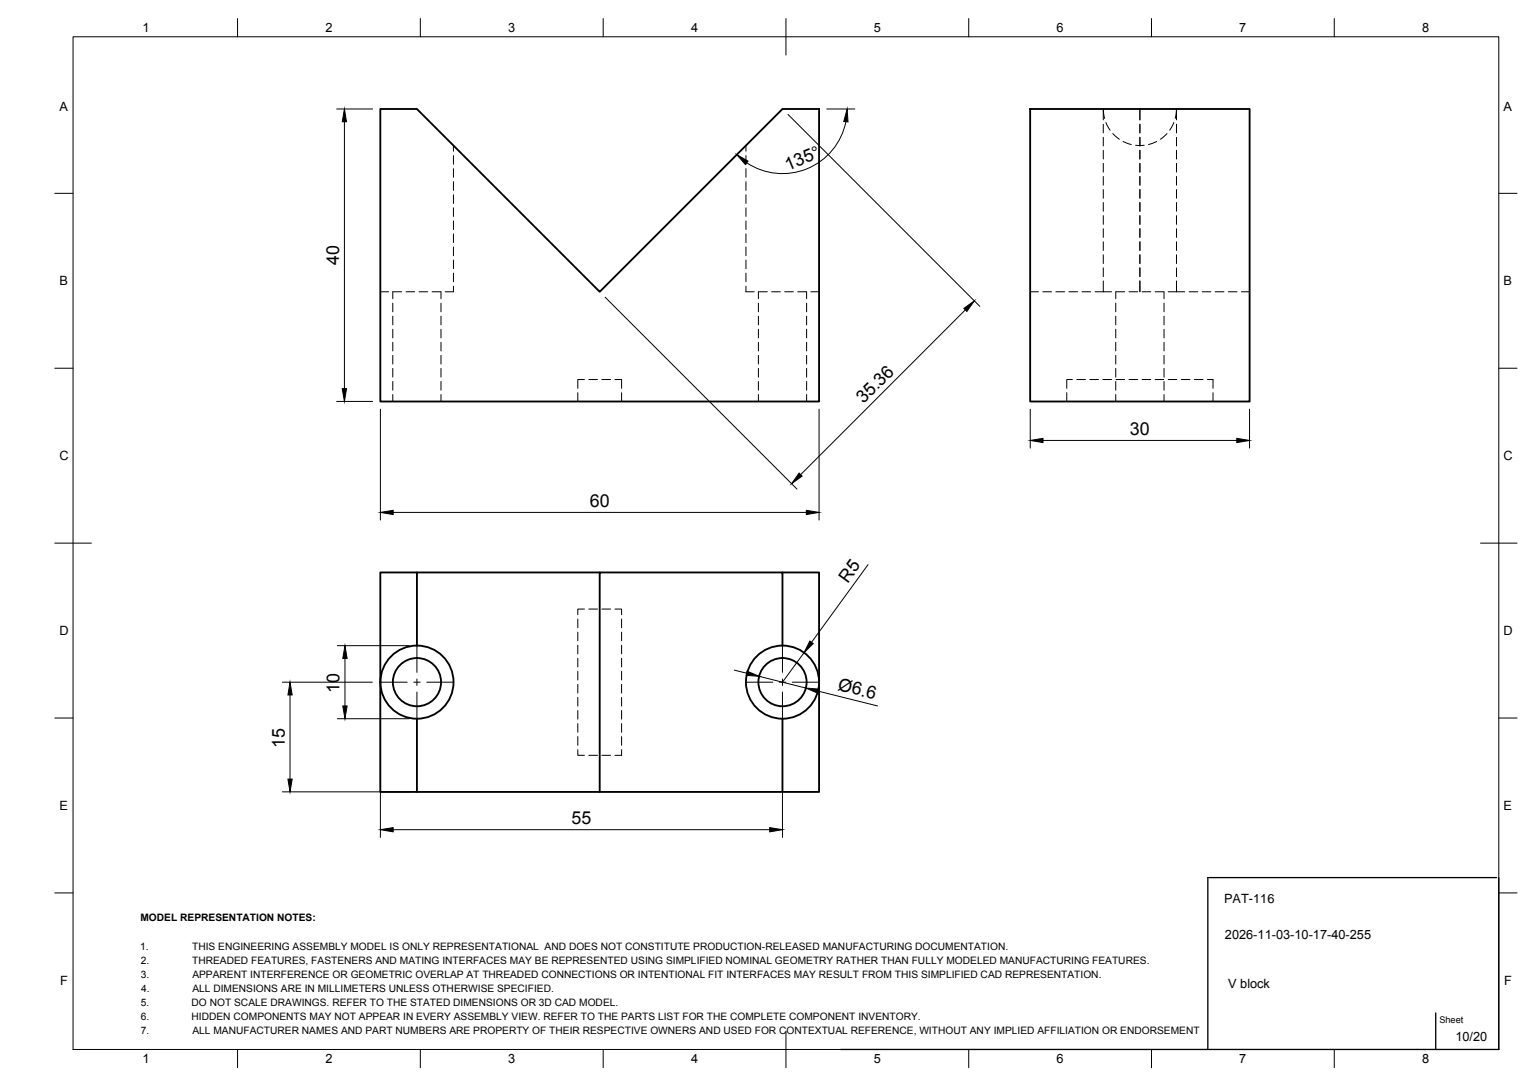
ISO-10303-21;
HEADER;
/* Generated by software containing ST-Developer
 * from STEP Tools, Inc. (www.steptools.com) 
 */

FILE_DESCRIPTION(
/* description */ ('V-block with clamp strap'),
/* implementation_level */ '2;1');

FILE_NAME(
/* name */ 'V block.step',
/* time_stamp */ '2026-10-27T10:50:53-07:00',
/* author */ (''),
/* organization */ (''),
/* preprocessor_version */ 'ST-DEVELOPER v20.2',
/* originating_system */ 'Autodesk Translation Framework v15.17.0.0',
/* authorisation */ '');

FILE_SCHEMA (('AUTOMOTIVE_DESIGN { 1 0 10303 214 3 1 1 }'));
ENDSEC;

DATA;
#10=MECHANICAL_DESIGN_GEOMETRIC_PRESENTATION_REPRESENTATION('',(#271),#7344);
#220=ELLIPSE('',#4506,0.707106781186547,0.5);
#221=ELLIPSE('',#4518,0.707106781186547,0.5);
#229=SHAPE_REPRESENTATION_RELATIONSHIP('SRR','None',#7447,#250);
#250=ADVANCED_BREP_SHAPE_REPRESENTATION('',(#292),#7326);
#271=STYLED_ITEM('',(#7610),#292);
#292=MANIFOLD_SOLID_BREP('Body1',#4153);
#339=FACE_BOUND('',#901,.T.);
#340=FACE_BOUND('',#904,.T.);
#341=FACE_BOUND('',#918,.T.);
#342=FACE_BOUND('',#919,.T.);
#343=FACE_BOUND('',#920,.T.);
#408=CIRCLE('',#4501,0.5);
#409=CIRCLE('',#4502,0.5);
#410=CIRCLE('',#4504,0.5);
#411=CIRCLE('',#4505,0.5);
#412=CIRCLE('',#4513,0.5);
#413=CIRCLE('',#4514,0.5);
#414=CIRCLE('',#4516,0.33);
#415=CIRCLE('',#4519,0.5);
#416=CIRCLE('',#4520,0.5);
#417=CIRCLE('',#4522,0.33);
#418=CIRCLE('',#4528,0.33);
#419=CIRCLE('',#4530,0.33);
#521=CYLINDRICAL_SURFACE('',#4500,0.5);
#522=CYLINDRICAL_SURFACE('',#4503,0.5);
#523=CYLINDRICAL_SURFACE('',#4512,0.5);
#524=CYLINDRICAL_SURFACE('',#4517,0.5);
#525=CYLINDRICAL_SURFACE('',#4527,0.33);
#526=CYLINDRICAL_SURFACE('',#4529,0.33);
#618=FACE_OUTER_BOUND('',#892,.T.);
#619=FACE_OUTER_BOUND('',#893,.T.);
#620=FACE_OUTER_BOUND('',#894,.T.);
#621=FACE_OUTER_BOUND('',#895,.T.);
#622=FACE_OUTER_BOUND('',#896,.T.);
#623=FACE_OUTER_BOUND('',#897,.T.);
#624=FACE_OUTER_BOUND('',#898,.T.);
#625=FACE_OUTER_BOUND('',#899,.T.);
#626=FACE_OUTER_BOUND('',#900,.T.);
#627=FACE_OUTER_BOUND('',#902,.T.);
#628=FACE_OUTER_BOUND('',#903,.T.);
#629=FACE_OUTER_BOUND('',#905,.T.);
#630=FACE_OUTER_BOUND('',#906,.T.);
#631=FACE_OUTER_BOUND('',#907,.T.);
#632=FACE_OUTER_BOUND('',#908,.T.);
#633=FACE_OUTER_BOUND('',#909,.T.);
#634=FACE_OUTER_BOUND('',#910,.T.);
#635=FACE_OUTER_BOUND('',#911,.T.);
#636=FACE_OUTER_BOUND('',#912,.T.);
#637=FACE_OUTER_BOUND('',#913,.T.);
#638=FACE_OUTER_BOUND('',#914,.T.);
#639=FACE_OUTER_BOUND('',#915,.T.);
#640=FACE_OUTER_BOUND('',#916,.T.);
#641=FACE_OUTER_BOUND('',#917,.T.);
#892=EDGE_LOOP('',(#2960,#2961,#2962,#2963));
#893=EDGE_LOOP('',(#2964,#2965,#2966,#2967,#2968));
#894=EDGE_LOOP('',(#2969,#2970,#2971,#2972));
#895=EDGE_LOOP('',(#2973,#2974,#2975,#2976));
#896=EDGE_LOOP('',(#2977,#2978,#2979,#2980));
#897=EDGE_LOOP('',(#2981,#2982,#2983,#2984));
#898=EDGE_LOOP('',(#2985,#2986,#2987,#2988));
#899=EDGE_LOOP('',(#2989,#2990,#2991,#2992));
#900=EDGE_LOOP('',(#2993,#2994));
#901=EDGE_LOOP('',(#2995));
#902=EDGE_LOOP('',(#2996,#2997,#2998,#2999,#3000));
#903=EDGE_LOOP('',(#3001,#3002));
#904=EDGE_LOOP('',(#3003));
#905=EDGE_LOOP('',(#3004,#3005,#3006,#3007,#3008,#3009));
#906=EDGE_LOOP('',(#3010,#3011,#3012,#3013));
#907=EDGE_LOOP('',(#3014,#3015,#3016,#3017,#3018,#3019));
#908=EDGE_LOOP('',(#3020,#3021,#3022,#3023));
#909=EDGE_LOOP('',(#3024,#3025,#3026,#3027));
#910=EDGE_LOOP('',(#3028,#3029,#3030,#3031));
#911=EDGE_LOOP('',(#3032,#3033,#3034,#3035));
#912=EDGE_LOOP('',(#3036,#3037,#3038,#3039));
#913=EDGE_LOOP('',(#3040,#3041,#3042,#3043,#3044,#3045,#3046));
#914=EDGE_LOOP('',(#3047,#3048,#3049,#3050,#3051,#3052,#3053));
#915=EDGE_LOOP('',(#3054,#3055,#3056,#3057,#3058,#3059,#3060));
#916=EDGE_LOOP('',(#3061,#3062,#3063,#3064,#3065,#3066,#3067));
#917=EDGE_LOOP('',(#3068,#3069,#3070,#3071));
#918=EDGE_LOOP('',(#3072,#3073,#3074,#3075));
#919=EDGE_LOOP('',(#3076));
#920=EDGE_LOOP('',(#3077));
#1213=LINE('',#6373,#1578);
#1214=LINE('',#6377,#1579);
#1215=LINE('',#6382,#1580);
#1216=LINE('',#6386,#1581);
#1217=LINE('',#6393,#1582);
#1218=LINE('',#6395,#1583);
#1219=LINE('',#6397,#1584);
#1220=LINE('',#6398,#1585);
#1221=LINE('',#6401,#1586);
#1222=LINE('',#6403,#1587);
#1223=LINE('',#6404,#1588);
#1224=LINE('',#6407,#1589);
#1225=LINE('',#6409,#1590);
#1226=LINE('',#6410,#1591);
#1227=LINE('',#6412,#1592);
#1228=LINE('',#6413,#1593);
#1229=LINE('',#6417,#1594);
#1230=LINE('',#6426,#1595);
#1231=LINE('',#6433,#1596);
#1232=LINE('',#6435,#1597);
#1233=LINE('',#6437,#1598);
#1234=LINE('',#6439,#1599);
#1235=LINE('',#6440,#1600);
#1236=LINE('',#6443,#1601);
#1237=LINE('',#6444,#1602);
#1238=LINE('',#6447,#1603);
#1239=LINE('',#6448,#1604);
#1240=LINE('',#6450,#1605);
#1241=LINE('',#6451,#1606);
#1242=LINE('',#6454,#1607);
#1243=LINE('',#6455,#1608);
#1244=LINE('',#6459,#1609);
#1245=LINE('',#6463,#1610);
#1246=LINE('',#6466,#1611);
#1247=LINE('',#6467,#1612);
#1248=LINE('',#6470,#1613);
#1249=LINE('',#6471,#1614);
#1250=LINE('',#6474,#1615);
#1251=LINE('',#6476,#1616);
#1252=LINE('',#6477,#1617);
#1253=LINE('',#6480,#1618);
#1254=LINE('',#6481,#1619);
#1255=LINE('',#6484,#1620);
#1256=LINE('',#6485,#1621);
#1257=LINE('',#6487,#1622);
#1578=VECTOR('',#5137,0.5);
#1579=VECTOR('',#5140,1.);
#1580=VECTOR('',#5145,0.5);
#1581=VECTOR('',#5148,1.);
#1582=VECTOR('',#5155,1.);
#1583=VECTOR('',#5156,1.);
#1584=VECTOR('',#5157,1.);
#1585=VECTOR('',#5158,1.);
#1586=VECTOR('',#5161,1.);
#1587=VECTOR('',#5162,1.);
#1588=VECTOR('',#5163,1.);
#1589=VECTOR('',#5166,1.);
#1590=VECTOR('',#5167,1.);
#1591=VECTOR('',#5168,1.);
#1592=VECTOR('',#5171,1.);
#1593=VECTOR('',#5172,1.);
#1594=VECTOR('',#5179,1.);
#1595=VECTOR('',#5192,1.);
#1596=VECTOR('',#5201,1.);
#1597=VECTOR('',#5202,1.);
#1598=VECTOR('',#5203,1.);
#1599=VECTOR('',#5204,1.);
#1600=VECTOR('',#5205,1.);
#1601=VECTOR('',#5208,1.);
#1602=VECTOR('',#5209,1.);
#1603=VECTOR('',#5212,1.);
#1604=VECTOR('',#5213,1.);
#1605=VECTOR('',#5214,1.);
#1606=VECTOR('',#5215,1.);
#1607=VECTOR('',#5218,1.);
#1608=VECTOR('',#5219,1.);
#1609=VECTOR('',#5224,0.33);
#1610=VECTOR('',#5229,0.33);
#1611=VECTOR('',#5232,1.);
#1612=VECTOR('',#5233,1.);
#1613=VECTOR('',#5236,1.);
#1614=VECTOR('',#5237,1.);
#1615=VECTOR('',#5240,1.);
#1616=VECTOR('',#5241,1.);
#1617=VECTOR('',#5242,1.);
#1618=VECTOR('',#5245,1.);
#1619=VECTOR('',#5246,1.);
#1620=VECTOR('',#5249,1.);
#1621=VECTOR('',#5250,1.);
#1622=VECTOR('',#5253,1.);
#1931=VERTEX_POINT('',#6371);
#1932=VERTEX_POINT('',#6372);
#1933=VERTEX_POINT('',#6374);
#1934=VERTEX_POINT('',#6376);
#1935=VERTEX_POINT('',#6380);
#1936=VERTEX_POINT('',#6381);
#1937=VERTEX_POINT('',#6383);
#1938=VERTEX_POINT('',#6385);
#1939=VERTEX_POINT('',#6387);
#1940=VERTEX_POINT('',#6391);
#1941=VERTEX_POINT('',#6392);
#1942=VERTEX_POINT('',#6394);
#1943=VERTEX_POINT('',#6396);
#1944=VERTEX_POINT('',#6400);
#1945=VERTEX_POINT('',#6402);
#1946=VERTEX_POINT('',#6406);
#1947=VERTEX_POINT('',#6408);
#1948=VERTEX_POINT('',#6420);
#1949=VERTEX_POINT('',#6423);
#1950=VERTEX_POINT('',#6429);
#1951=VERTEX_POINT('',#6432);
#1952=VERTEX_POINT('',#6434);
#1953=VERTEX_POINT('',#6436);
#1954=VERTEX_POINT('',#6438);
#1955=VERTEX_POINT('',#6442);
#1956=VERTEX_POINT('',#6446);
#1957=VERTEX_POINT('',#6449);
#1958=VERTEX_POINT('',#6453);
#1959=VERTEX_POINT('',#6457);
#1960=VERTEX_POINT('',#6461);
#1961=VERTEX_POINT('',#6465);
#1962=VERTEX_POINT('',#6469);
#1963=VERTEX_POINT('',#6473);
#1964=VERTEX_POINT('',#6475);
#1965=VERTEX_POINT('',#6479);
#1966=VERTEX_POINT('',#6483);
#2306=EDGE_CURVE('',#1931,#1932,#1213,.T.);
#2307=EDGE_CURVE('',#1933,#1931,#408,.T.);
#2308=EDGE_CURVE('',#1933,#1934,#1214,.T.);
#2309=EDGE_CURVE('',#1932,#1934,#409,.T.);
#2310=EDGE_CURVE('',#1935,#1936,#1215,.T.);
#2311=EDGE_CURVE('',#1937,#1935,#410,.T.);
#2312=EDGE_CURVE('',#1937,#1938,#1216,.T.);
#2313=EDGE_CURVE('',#1939,#1938,#411,.T.);
#2314=EDGE_CURVE('',#1936,#1939,#220,.T.);
#2315=EDGE_CURVE('',#1940,#1941,#1217,.T.);
#2316=EDGE_CURVE('',#1940,#1942,#1218,.T.);
#2317=EDGE_CURVE('',#1942,#1943,#1219,.T.);
#2318=EDGE_CURVE('',#1941,#1943,#1220,.T.);
#2319=EDGE_CURVE('',#1941,#1944,#1221,.T.);
#2320=EDGE_CURVE('',#1943,#1945,#1222,.T.);
#2321=EDGE_CURVE('',#1944,#1945,#1223,.T.);
#2322=EDGE_CURVE('',#1944,#1946,#1224,.T.);
#2323=EDGE_CURVE('',#1945,#1947,#1225,.T.);
#2324=EDGE_CURVE('',#1946,#1947,#1226,.T.);
#2325=EDGE_CURVE('',#1946,#1940,#1227,.T.);
#2326=EDGE_CURVE('',#1947,#1942,#1228,.T.);
#2327=EDGE_CURVE('',#1938,#1936,#412,.T.);
#2328=EDGE_CURVE('',#1937,#1938,#1229,.T.);
#2329=EDGE_CURVE('',#1935,#1937,#413,.T.);
#2330=EDGE_CURVE('',#1948,#1948,#414,.T.);
#2331=EDGE_CURVE('',#1949,#1932,#221,.T.);
#2332=EDGE_CURVE('',#1934,#1949,#415,.T.);
#2333=EDGE_CURVE('',#1933,#1934,#1230,.T.);
#2334=EDGE_CURVE('',#1931,#1933,#416,.T.);
#2335=EDGE_CURVE('',#1950,#1950,#417,.T.);
#2336=EDGE_CURVE('',#1951,#1939,#1231,.T.);
#2337=EDGE_CURVE('',#1952,#1951,#1232,.T.);
#2338=EDGE_CURVE('',#1953,#1952,#1233,.T.);
#2339=EDGE_CURVE('',#1954,#1953,#1234,.T.);
#2340=EDGE_CURVE('',#1936,#1954,#1235,.T.);
#2341=EDGE_CURVE('',#1938,#1955,#1236,.T.);
#2342=EDGE_CURVE('',#1955,#1951,#1237,.T.);
#2343=EDGE_CURVE('',#1956,#1932,#1238,.T.);
#2344=EDGE_CURVE('',#1953,#1956,#1239,.T.);
#2345=EDGE_CURVE('',#1957,#1952,#1240,.T.);
#2346=EDGE_CURVE('',#1949,#1957,#1241,.T.);
#2347=EDGE_CURVE('',#1934,#1958,#1242,.T.);
#2348=EDGE_CURVE('',#1958,#1956,#1243,.T.);
#2349=EDGE_CURVE('',#1959,#1959,#418,.T.);
#2350=EDGE_CURVE('',#1959,#1948,#1244,.T.);
#2351=EDGE_CURVE('',#1960,#1960,#419,.T.);
#2352=EDGE_CURVE('',#1960,#1950,#1245,.T.);
#2353=EDGE_CURVE('',#1954,#1961,#1246,.T.);
#2354=EDGE_CURVE('',#1961,#1938,#1247,.T.);
#2355=EDGE_CURVE('',#1957,#1962,#1248,.T.);
#2356=EDGE_CURVE('',#1962,#1934,#1249,.T.);
#2357=EDGE_CURVE('',#1963,#1958,#1250,.T.);
#2358=EDGE_CURVE('',#1963,#1964,#1251,.T.);
#2359=EDGE_CURVE('',#1964,#1961,#1252,.T.);
#2360=EDGE_CURVE('',#1965,#1963,#1253,.T.);
#2361=EDGE_CURVE('',#1965,#1962,#1254,.T.);
#2362=EDGE_CURVE('',#1966,#1955,#1255,.T.);
#2363=EDGE_CURVE('',#1966,#1965,#1256,.T.);
#2364=EDGE_CURVE('',#1964,#1966,#1257,.T.);
#2960=ORIENTED_EDGE('',*,*,#2306,.F.);
#2961=ORIENTED_EDGE('',*,*,#2307,.F.);
#2962=ORIENTED_EDGE('',*,*,#2308,.T.);
#2963=ORIENTED_EDGE('',*,*,#2309,.F.);
#2964=ORIENTED_EDGE('',*,*,#2310,.F.);
#2965=ORIENTED_EDGE('',*,*,#2311,.F.);
#2966=ORIENTED_EDGE('',*,*,#2312,.T.);
#2967=ORIENTED_EDGE('',*,*,#2313,.F.);
#2968=ORIENTED_EDGE('',*,*,#2314,.F.);
#2969=ORIENTED_EDGE('',*,*,#2315,.F.);
#2970=ORIENTED_EDGE('',*,*,#2316,.T.);
#2971=ORIENTED_EDGE('',*,*,#2317,.T.);
#2972=ORIENTED_EDGE('',*,*,#2318,.F.);
#2973=ORIENTED_EDGE('',*,*,#2319,.F.);
#2974=ORIENTED_EDGE('',*,*,#2318,.T.);
#2975=ORIENTED_EDGE('',*,*,#2320,.T.);
#2976=ORIENTED_EDGE('',*,*,#2321,.F.);
#2977=ORIENTED_EDGE('',*,*,#2322,.F.);
#2978=ORIENTED_EDGE('',*,*,#2321,.T.);
#2979=ORIENTED_EDGE('',*,*,#2323,.T.);
#2980=ORIENTED_EDGE('',*,*,#2324,.F.);
#2981=ORIENTED_EDGE('',*,*,#2325,.F.);
#2982=ORIENTED_EDGE('',*,*,#2324,.T.);
#2983=ORIENTED_EDGE('',*,*,#2326,.T.);
#2984=ORIENTED_EDGE('',*,*,#2316,.F.);
#2985=ORIENTED_EDGE('',*,*,#2326,.F.);
#2986=ORIENTED_EDGE('',*,*,#2323,.F.);
#2987=ORIENTED_EDGE('',*,*,#2320,.F.);
#2988=ORIENTED_EDGE('',*,*,#2317,.F.);
#2989=ORIENTED_EDGE('',*,*,#2310,.T.);
#2990=ORIENTED_EDGE('',*,*,#2327,.F.);
#2991=ORIENTED_EDGE('',*,*,#2328,.F.);
#2992=ORIENTED_EDGE('',*,*,#2329,.F.);
#2993=ORIENTED_EDGE('',*,*,#2311,.T.);
#2994=ORIENTED_EDGE('',*,*,#2329,.T.);
#2995=ORIENTED_EDGE('',*,*,#2330,.F.);
#2996=ORIENTED_EDGE('',*,*,#2306,.T.);
#2997=ORIENTED_EDGE('',*,*,#2331,.F.);
#2998=ORIENTED_EDGE('',*,*,#2332,.F.);
#2999=ORIENTED_EDGE('',*,*,#2333,.F.);
#3000=ORIENTED_EDGE('',*,*,#2334,.F.);
#3001=ORIENTED_EDGE('',*,*,#2307,.T.);
#3002=ORIENTED_EDGE('',*,*,#2334,.T.);
#3003=ORIENTED_EDGE('',*,*,#2335,.F.);
#3004=ORIENTED_EDGE('',*,*,#2314,.T.);
#3005=ORIENTED_EDGE('',*,*,#2336,.F.);
#3006=ORIENTED_EDGE('',*,*,#2337,.F.);
#3007=ORIENTED_EDGE('',*,*,#2338,.F.);
#3008=ORIENTED_EDGE('',*,*,#2339,.F.);
#3009=ORIENTED_EDGE('',*,*,#2340,.F.);
#3010=ORIENTED_EDGE('',*,*,#2313,.T.);
#3011=ORIENTED_EDGE('',*,*,#2341,.T.);
#3012=ORIENTED_EDGE('',*,*,#2342,.T.);
#3013=ORIENTED_EDGE('',*,*,#2336,.T.);
#3014=ORIENTED_EDGE('',*,*,#2331,.T.);
#3015=ORIENTED_EDGE('',*,*,#2343,.F.);
#3016=ORIENTED_EDGE('',*,*,#2344,.F.);
#3017=ORIENTED_EDGE('',*,*,#2338,.T.);
#3018=ORIENTED_EDGE('',*,*,#2345,.F.);
#3019=ORIENTED_EDGE('',*,*,#2346,.F.);
#3020=ORIENTED_EDGE('',*,*,#2309,.T.);
#3021=ORIENTED_EDGE('',*,*,#2347,.T.);
#3022=ORIENTED_EDGE('',*,*,#2348,.T.);
#3023=ORIENTED_EDGE('',*,*,#2343,.T.);
#3024=ORIENTED_EDGE('',*,*,#2349,.F.);
#3025=ORIENTED_EDGE('',*,*,#2350,.T.);
#3026=ORIENTED_EDGE('',*,*,#2330,.T.);
#3027=ORIENTED_EDGE('',*,*,#2350,.F.);
#3028=ORIENTED_EDGE('',*,*,#2351,.F.);
#3029=ORIENTED_EDGE('',*,*,#2352,.T.);
#3030=ORIENTED_EDGE('',*,*,#2335,.T.);
#3031=ORIENTED_EDGE('',*,*,#2352,.F.);
#3032=ORIENTED_EDGE('',*,*,#2327,.T.);
#3033=ORIENTED_EDGE('',*,*,#2340,.T.);
#3034=ORIENTED_EDGE('',*,*,#2353,.T.);
#3035=ORIENTED_EDGE('',*,*,#2354,.T.);
#3036=ORIENTED_EDGE('',*,*,#2332,.T.);
#3037=ORIENTED_EDGE('',*,*,#2346,.T.);
#3038=ORIENTED_EDGE('',*,*,#2355,.T.);
#3039=ORIENTED_EDGE('',*,*,#2356,.T.);
#3040=ORIENTED_EDGE('',*,*,#2339,.T.);
#3041=ORIENTED_EDGE('',*,*,#2344,.T.);
#3042=ORIENTED_EDGE('',*,*,#2348,.F.);
#3043=ORIENTED_EDGE('',*,*,#2357,.F.);
#3044=ORIENTED_EDGE('',*,*,#2358,.T.);
#3045=ORIENTED_EDGE('',*,*,#2359,.T.);
#3046=ORIENTED_EDGE('',*,*,#2353,.F.);
#3047=ORIENTED_EDGE('',*,*,#2360,.T.);
#3048=ORIENTED_EDGE('',*,*,#2357,.T.);
#3049=ORIENTED_EDGE('',*,*,#2347,.F.);
#3050=ORIENTED_EDGE('',*,*,#2308,.F.);
#3051=ORIENTED_EDGE('',*,*,#2333,.T.);
#3052=ORIENTED_EDGE('',*,*,#2356,.F.);
#3053=ORIENTED_EDGE('',*,*,#2361,.F.);
#3054=ORIENTED_EDGE('',*,*,#2337,.T.);
#3055=ORIENTED_EDGE('',*,*,#2342,.F.);
#3056=ORIENTED_EDGE('',*,*,#2362,.F.);
#3057=ORIENTED_EDGE('',*,*,#2363,.T.);
#3058=ORIENTED_EDGE('',*,*,#2361,.T.);
#3059=ORIENTED_EDGE('',*,*,#2355,.F.);
#3060=ORIENTED_EDGE('',*,*,#2345,.T.);
#3061=ORIENTED_EDGE('',*,*,#2364,.T.);
#3062=ORIENTED_EDGE('',*,*,#2362,.T.);
#3063=ORIENTED_EDGE('',*,*,#2341,.F.);
#3064=ORIENTED_EDGE('',*,*,#2312,.F.);
#3065=ORIENTED_EDGE('',*,*,#2328,.T.);
#3066=ORIENTED_EDGE('',*,*,#2354,.F.);
#3067=ORIENTED_EDGE('',*,*,#2359,.F.);
#3068=ORIENTED_EDGE('',*,*,#2358,.F.);
#3069=ORIENTED_EDGE('',*,*,#2360,.F.);
#3070=ORIENTED_EDGE('',*,*,#2363,.F.);
#3071=ORIENTED_EDGE('',*,*,#2364,.F.);
#3072=ORIENTED_EDGE('',*,*,#2322,.T.);
#3073=ORIENTED_EDGE('',*,*,#2325,.T.);
#3074=ORIENTED_EDGE('',*,*,#2315,.T.);
#3075=ORIENTED_EDGE('',*,*,#2319,.T.);
#3076=ORIENTED_EDGE('',*,*,#2349,.T.);
#3077=ORIENTED_EDGE('',*,*,#2351,.T.);
#3780=PLANE('',#4507);
#3781=PLANE('',#4508);
#3782=PLANE('',#4509);
#3783=PLANE('',#4510);
#3784=PLANE('',#4511);
#3785=PLANE('',#4515);
#3786=PLANE('',#4521);
#3787=PLANE('',#4523);
#3788=PLANE('',#4524);
#3789=PLANE('',#4525);
#3790=PLANE('',#4526);
#3791=PLANE('',#4531);
#3792=PLANE('',#4532);
#3793=PLANE('',#4533);
#3794=PLANE('',#4534);
#3795=PLANE('',#4535);
#3796=PLANE('',#4536);
#3797=PLANE('',#4537);
#3964=ADVANCED_FACE('',(#618),#521,.F.);
#3965=ADVANCED_FACE('',(#619),#522,.F.);
#3966=ADVANCED_FACE('',(#620),#3780,.F.);
#3967=ADVANCED_FACE('',(#621),#3781,.F.);
#3968=ADVANCED_FACE('',(#622),#3782,.F.);
#3969=ADVANCED_FACE('',(#623),#3783,.F.);
#3970=ADVANCED_FACE('',(#624),#3784,.F.);
#3971=ADVANCED_FACE('',(#625),#523,.F.);
#3972=ADVANCED_FACE('',(#626,#339),#3785,.T.);
#3973=ADVANCED_FACE('',(#627),#524,.F.);
#3974=ADVANCED_FACE('',(#628,#340),#3786,.T.);
#3975=ADVANCED_FACE('',(#629),#3787,.F.);
#3976=ADVANCED_FACE('',(#630),#3788,.T.);
#3977=ADVANCED_FACE('',(#631),#3789,.F.);
#3978=ADVANCED_FACE('',(#632),#3790,.T.);
#3979=ADVANCED_FACE('',(#633),#525,.F.);
#3980=ADVANCED_FACE('',(#634),#526,.F.);
#3981=ADVANCED_FACE('',(#635),#3791,.T.);
#3982=ADVANCED_FACE('',(#636),#3792,.T.);
#3983=ADVANCED_FACE('',(#637),#3793,.T.);
#3984=ADVANCED_FACE('',(#638),#3794,.T.);
#3985=ADVANCED_FACE('',(#639),#3795,.T.);
#3986=ADVANCED_FACE('',(#640),#3796,.T.);
#3987=ADVANCED_FACE('',(#641,#341,#342,#343),#3797,.F.);
#4153=CLOSED_SHELL('',(#3964,#3965,#3966,#3967,#3968,#3969,#3970,#3971,
#3972,#3973,#3974,#3975,#3976,#3977,#3978,#3979,#3980,#3981,#3982,#3983,
#3984,#3985,#3986,#3987));
#4499=AXIS2_PLACEMENT_3D('',#6369,#5133,#5134);
#4500=AXIS2_PLACEMENT_3D('',#6370,#5135,#5136);
#4501=AXIS2_PLACEMENT_3D('',#6375,#5138,#5139);
#4502=AXIS2_PLACEMENT_3D('',#6378,#5141,#5142);
#4503=AXIS2_PLACEMENT_3D('',#6379,#5143,#5144);
#4504=AXIS2_PLACEMENT_3D('',#6384,#5146,#5147);
#4505=AXIS2_PLACEMENT_3D('',#6388,#5149,#5150);
#4506=AXIS2_PLACEMENT_3D('',#6389,#5151,#5152);
#4507=AXIS2_PLACEMENT_3D('',#6390,#5153,#5154);
#4508=AXIS2_PLACEMENT_3D('',#6399,#5159,#5160);
#4509=AXIS2_PLACEMENT_3D('',#6405,#5164,#5165);
#4510=AXIS2_PLACEMENT_3D('',#6411,#5169,#5170);
#4511=AXIS2_PLACEMENT_3D('',#6414,#5173,#5174);
#4512=AXIS2_PLACEMENT_3D('',#6415,#5175,#5176);
#4513=AXIS2_PLACEMENT_3D('',#6416,#5177,#5178);
#4514=AXIS2_PLACEMENT_3D('',#6418,#5180,#5181);
#4515=AXIS2_PLACEMENT_3D('',#6419,#5182,#5183);
#4516=AXIS2_PLACEMENT_3D('',#6421,#5184,#5185);
#4517=AXIS2_PLACEMENT_3D('',#6422,#5186,#5187);
#4518=AXIS2_PLACEMENT_3D('',#6424,#5188,#5189);
#4519=AXIS2_PLACEMENT_3D('',#6425,#5190,#5191);
#4520=AXIS2_PLACEMENT_3D('',#6427,#5193,#5194);
#4521=AXIS2_PLACEMENT_3D('',#6428,#5195,#5196);
#4522=AXIS2_PLACEMENT_3D('',#6430,#5197,#5198);
#4523=AXIS2_PLACEMENT_3D('',#6431,#5199,#5200);
#4524=AXIS2_PLACEMENT_3D('',#6441,#5206,#5207);
#4525=AXIS2_PLACEMENT_3D('',#6445,#5210,#5211);
#4526=AXIS2_PLACEMENT_3D('',#6452,#5216,#5217);
#4527=AXIS2_PLACEMENT_3D('',#6456,#5220,#5221);
#4528=AXIS2_PLACEMENT_3D('',#6458,#5222,#5223);
#4529=AXIS2_PLACEMENT_3D('',#6460,#5225,#5226);
#4530=AXIS2_PLACEMENT_3D('',#6462,#5227,#5228);
#4531=AXIS2_PLACEMENT_3D('',#6464,#5230,#5231);
#4532=AXIS2_PLACEMENT_3D('',#6468,#5234,#5235);
#4533=AXIS2_PLACEMENT_3D('',#6472,#5238,#5239);
#4534=AXIS2_PLACEMENT_3D('',#6478,#5243,#5244);
#4535=AXIS2_PLACEMENT_3D('',#6482,#5247,#5248);
#4536=AXIS2_PLACEMENT_3D('',#6486,#5251,#5252);
#4537=AXIS2_PLACEMENT_3D('',#6488,#5254,#5255);
#5133=DIRECTION('axis',(0.,0.,1.));
#5134=DIRECTION('refdir',(1.,0.,0.));
#5135=DIRECTION('center_axis',(0.,0.,1.));
#5136=DIRECTION('ref_axis',(1.,0.,0.));
#5137=DIRECTION('',(0.,0.,1.));
#5138=DIRECTION('center_axis',(0.,0.,1.));
#5139=DIRECTION('ref_axis',(1.,0.,0.));
#5140=DIRECTION('',(0.,0.,1.));
#5141=DIRECTION('center_axis',(0.,0.,-1.));
#5142=DIRECTION('ref_axis',(1.,0.,0.));
#5143=DIRECTION('center_axis',(0.,0.,1.));
#5144=DIRECTION('ref_axis',(1.,0.,0.));
#5145=DIRECTION('',(0.,0.,1.));
#5146=DIRECTION('center_axis',(0.,0.,1.));
#5147=DIRECTION('ref_axis',(1.,0.,0.));
#5148=DIRECTION('',(0.,0.,1.));
#5149=DIRECTION('center_axis',(0.,0.,-1.));
#5150=DIRECTION('ref_axis',(1.,0.,0.));
#5151=DIRECTION('center_axis',(0.,-0.707106781186547,-0.707106781186548));
#5152=DIRECTION('ref_axis',(0.,0.707106781186548,-0.707106781186547));
#5153=DIRECTION('center_axis',(0.,-1.,0.));
#5154=DIRECTION('ref_axis',(1.,0.,0.));
#5155=DIRECTION('',(1.,0.,0.));
#5156=DIRECTION('',(0.,0.,1.));
#5157=DIRECTION('',(1.,0.,0.));
#5158=DIRECTION('',(0.,0.,1.));
#5159=DIRECTION('center_axis',(1.,0.,0.));
#5160=DIRECTION('ref_axis',(0.,1.,0.));
#5161=DIRECTION('',(0.,1.,0.));
#5162=DIRECTION('',(0.,1.,0.));
#5163=DIRECTION('',(0.,0.,1.));
#5164=DIRECTION('center_axis',(0.,1.,0.));
#5165=DIRECTION('ref_axis',(-1.,0.,0.));
#5166=DIRECTION('',(-1.,0.,0.));
#5167=DIRECTION('',(-1.,0.,0.));
#5168=DIRECTION('',(0.,0.,1.));
#5169=DIRECTION('center_axis',(-1.,0.,0.));
#5170=DIRECTION('ref_axis',(0.,-1.,0.));
#5171=DIRECTION('',(0.,-1.,0.));
#5172=DIRECTION('',(0.,-1.,0.));
#5173=DIRECTION('center_axis',(0.,0.,1.));
#5174=DIRECTION('ref_axis',(1.,0.,0.));
#5175=DIRECTION('center_axis',(0.,0.,1.));
#5176=DIRECTION('ref_axis',(1.,0.,0.));
#5177=DIRECTION('center_axis',(0.,0.,-1.));
#5178=DIRECTION('ref_axis',(1.,0.,0.));
#5179=DIRECTION('',(0.,0.,1.));
#5180=DIRECTION('center_axis',(0.,0.,1.));
#5181=DIRECTION('ref_axis',(1.,0.,0.));
#5182=DIRECTION('center_axis',(0.,0.,1.));
#5183=DIRECTION('ref_axis',(1.,0.,0.));
#5184=DIRECTION('center_axis',(0.,0.,1.));
#5185=DIRECTION('ref_axis',(1.,0.,0.));
#5186=DIRECTION('center_axis',(0.,0.,1.));
#5187=DIRECTION('ref_axis',(1.,0.,0.));
#5188=DIRECTION('center_axis',(0.,0.707106781186547,-0.707106781186548));
#5189=DIRECTION('ref_axis',(0.,0.707106781186548,0.707106781186547));
#5190=DIRECTION('center_axis',(0.,0.,-1.));
#5191=DIRECTION('ref_axis',(1.,0.,0.));
#5192=DIRECTION('',(0.,0.,1.));
#5193=DIRECTION('center_axis',(0.,0.,1.));
#5194=DIRECTION('ref_axis',(1.,0.,0.));
#5195=DIRECTION('center_axis',(0.,0.,1.));
#5196=DIRECTION('ref_axis',(1.,0.,0.));
#5197=DIRECTION('center_axis',(0.,0.,1.));
#5198=DIRECTION('ref_axis',(1.,0.,0.));
#5199=DIRECTION('center_axis',(0.,-0.707106781186547,-0.707106781186548));
#5200=DIRECTION('ref_axis',(0.,0.707106781186548,-0.707106781186547));
#5201=DIRECTION('',(-1.,0.,0.));
#5202=DIRECTION('',(0.,-0.707106781186548,0.707106781186547));
#5203=DIRECTION('',(1.,0.,0.));
#5204=DIRECTION('',(0.,0.707106781186548,-0.707106781186547));
#5205=DIRECTION('',(-1.,0.,0.));
#5206=DIRECTION('center_axis',(0.,0.,1.));
#5207=DIRECTION('ref_axis',(1.,0.,0.));
#5208=DIRECTION('',(1.,0.,0.));
#5209=DIRECTION('',(0.,1.,0.));
#5210=DIRECTION('center_axis',(0.,0.707106781186547,-0.707106781186548));
#5211=DIRECTION('ref_axis',(0.,0.707106781186548,0.707106781186547));
#5212=DIRECTION('',(1.,0.,0.));
#5213=DIRECTION('',(0.,0.707106781186548,0.707106781186547));
#5214=DIRECTION('',(0.,-0.707106781186548,-0.707106781186547));
#5215=DIRECTION('',(1.,0.,0.));
#5216=DIRECTION('center_axis',(0.,0.,1.));
#5217=DIRECTION('ref_axis',(1.,0.,0.));
#5218=DIRECTION('',(-1.,0.,0.));
#5219=DIRECTION('',(0.,-1.,0.));
#5220=DIRECTION('center_axis',(0.,0.,1.));
#5221=DIRECTION('ref_axis',(1.,0.,0.));
#5222=DIRECTION('center_axis',(0.,0.,1.));
#5223=DIRECTION('ref_axis',(1.,0.,0.));
#5224=DIRECTION('',(0.,0.,1.));
#5225=DIRECTION('center_axis',(0.,0.,1.));
#5226=DIRECTION('ref_axis',(1.,0.,0.));
#5227=DIRECTION('center_axis',(0.,0.,1.));
#5228=DIRECTION('ref_axis',(1.,0.,0.));
#5229=DIRECTION('',(0.,0.,1.));
#5230=DIRECTION('center_axis',(0.,0.,1.));
#5231=DIRECTION('ref_axis',(1.,0.,0.));
#5232=DIRECTION('',(0.,-1.,0.));
#5233=DIRECTION('',(1.,0.,0.));
#5234=DIRECTION('center_axis',(0.,0.,1.));
#5235=DIRECTION('ref_axis',(1.,0.,0.));
#5236=DIRECTION('',(0.,1.,0.));
#5237=DIRECTION('',(-1.,0.,0.));
#5238=DIRECTION('center_axis',(-1.,0.,0.));
#5239=DIRECTION('ref_axis',(0.,-1.,0.));
#5240=DIRECTION('',(0.,0.,1.));
#5241=DIRECTION('',(0.,-1.,0.));
#5242=DIRECTION('',(0.,0.,1.));
#5243=DIRECTION('center_axis',(0.,1.,0.));
#5244=DIRECTION('ref_axis',(-1.,0.,0.));
#5245=DIRECTION('',(-1.,0.,0.));
#5246=DIRECTION('',(0.,0.,1.));
#5247=DIRECTION('center_axis',(1.,0.,0.));
#5248=DIRECTION('ref_axis',(0.,1.,0.));
#5249=DIRECTION('',(0.,0.,1.));
#5250=DIRECTION('',(0.,1.,0.));
#5251=DIRECTION('center_axis',(0.,-1.,0.));
#5252=DIRECTION('ref_axis',(1.,0.,0.));
#5253=DIRECTION('',(1.,0.,0.));
#5254=DIRECTION('center_axis',(0.,0.,1.));
#5255=DIRECTION('ref_axis',(1.,0.,0.));
#6369=CARTESIAN_POINT('',(0.,0.,0.));
#6370=CARTESIAN_POINT('Origin',(6.5,2.5,2.5));
#6371=CARTESIAN_POINT('',(6.,2.5,2.5));
#6372=CARTESIAN_POINT('',(6.,2.5,5.));
#6373=CARTESIAN_POINT('',(6.,2.5,2.5));
#6374=CARTESIAN_POINT('',(6.5,3.,2.5));
#6375=CARTESIAN_POINT('Origin',(6.5,2.5,2.5));
#6376=CARTESIAN_POINT('',(6.5,3.,5.));
#6377=CARTESIAN_POINT('',(6.5,3.,2.5));
#6378=CARTESIAN_POINT('Origin',(6.5,2.5,5.));
#6379=CARTESIAN_POINT('Origin',(6.5,-2.5,2.5));
#6380=CARTESIAN_POINT('',(6.,-2.5,2.5));
#6381=CARTESIAN_POINT('',(6.,-2.5,5.));
#6382=CARTESIAN_POINT('',(6.,-2.5,2.5));
#6383=CARTESIAN_POINT('',(6.5,-3.,2.5));
#6384=CARTESIAN_POINT('Origin',(6.5,-2.5,2.5));
#6385=CARTESIAN_POINT('',(6.5,-3.,5.));
#6386=CARTESIAN_POINT('',(6.5,-3.,2.5));
#6387=CARTESIAN_POINT('',(7.,-2.5,5.));
#6388=CARTESIAN_POINT('Origin',(6.5,-2.5,5.));
#6389=CARTESIAN_POINT('Origin',(6.5,-2.5,5.));
#6390=CARTESIAN_POINT('Origin',(5.5,-0.3,0.9));
#6391=CARTESIAN_POINT('',(5.5,-0.3,1.));
#6392=CARTESIAN_POINT('',(7.5,-0.3,1.));
#6393=CARTESIAN_POINT('',(6.,-0.3,1.));
#6394=CARTESIAN_POINT('',(5.5,-0.3,1.3));
#6395=CARTESIAN_POINT('',(5.5,-0.3,0.9));
#6396=CARTESIAN_POINT('',(7.5,-0.3,1.3));
#6397=CARTESIAN_POINT('',(5.5,-0.3,1.3));
#6398=CARTESIAN_POINT('',(7.5,-0.3,0.9));
#6399=CARTESIAN_POINT('Origin',(7.5,-0.3,0.9));
#6400=CARTESIAN_POINT('',(7.5,0.3,1.));
#6401=CARTESIAN_POINT('',(7.5,-0.15,1.));
#6402=CARTESIAN_POINT('',(7.5,0.3,1.3));
#6403=CARTESIAN_POINT('',(7.5,-0.3,1.3));
#6404=CARTESIAN_POINT('',(7.5,0.3,0.9));
#6405=CARTESIAN_POINT('Origin',(7.5,0.3,0.9));
#6406=CARTESIAN_POINT('',(5.5,0.3,1.));
#6407=CARTESIAN_POINT('',(7.,0.3,1.));
#6408=CARTESIAN_POINT('',(5.5,0.3,1.3));
#6409=CARTESIAN_POINT('',(7.5,0.3,1.3));
#6410=CARTESIAN_POINT('',(5.5,0.3,0.9));
#6411=CARTESIAN_POINT('Origin',(5.5,0.3,0.9));
#6412=CARTESIAN_POINT('',(5.5,0.15,1.));
#6413=CARTESIAN_POINT('',(5.5,0.3,1.3));
#6414=CARTESIAN_POINT('Origin',(6.5,0.,1.3));
#6415=CARTESIAN_POINT('Origin',(6.5,-2.5,2.5));
#6416=CARTESIAN_POINT('Origin',(6.5,-2.5,5.));
#6417=CARTESIAN_POINT('',(6.5,-3.,2.5));
#6418=CARTESIAN_POINT('Origin',(6.5,-2.5,2.5));
#6419=CARTESIAN_POINT('Origin',(6.5,-2.5,2.5));
#6420=CARTESIAN_POINT('',(6.17,-2.5,2.5));
#6421=CARTESIAN_POINT('Origin',(6.5,-2.5,2.5));
#6422=CARTESIAN_POINT('Origin',(6.5,2.5,2.5));
#6423=CARTESIAN_POINT('',(7.,2.5,5.));
#6424=CARTESIAN_POINT('Origin',(6.5,2.5,5.));
#6425=CARTESIAN_POINT('Origin',(6.5,2.5,5.));
#6426=CARTESIAN_POINT('',(6.5,3.,2.5));
#6427=CARTESIAN_POINT('Origin',(6.5,2.5,2.5));
#6428=CARTESIAN_POINT('Origin',(6.5,2.5,2.5));
#6429=CARTESIAN_POINT('',(6.17,2.5,2.5));
#6430=CARTESIAN_POINT('Origin',(6.5,2.5,2.5));
#6431=CARTESIAN_POINT('Origin',(4.9,-2.6,5.1));
#6432=CARTESIAN_POINT('',(8.,-2.5,5.));
#6433=CARTESIAN_POINT('',(5.7,-2.5,5.));
#6434=CARTESIAN_POINT('',(8.,0.,2.5));
#6435=CARTESIAN_POINT('',(8.,-1.675,4.175));
#6436=CARTESIAN_POINT('',(5.,0.,2.5));
#6437=CARTESIAN_POINT('',(4.9,0.,2.5));
#6438=CARTESIAN_POINT('',(5.,-2.5,5.));
#6439=CARTESIAN_POINT('',(5.,-0.175,2.675));
#6440=CARTESIAN_POINT('',(5.7,-2.5,5.));
#6441=CARTESIAN_POINT('Origin',(6.5,0.,5.));
#6442=CARTESIAN_POINT('',(8.,-3.,5.));
#6443=CARTESIAN_POINT('',(5.,-3.,5.));
#6444=CARTESIAN_POINT('',(8.,-3.,5.));
#6445=CARTESIAN_POINT('Origin',(4.9,0.,2.5));
#6446=CARTESIAN_POINT('',(5.,2.5,5.));
#6447=CARTESIAN_POINT('',(5.7,2.5,5.));
#6448=CARTESIAN_POINT('',(5.,0.375,2.875));
#6449=CARTESIAN_POINT('',(8.,2.5,5.));
#6450=CARTESIAN_POINT('',(8.,-1.125,1.375));
#6451=CARTESIAN_POINT('',(5.7,2.5,5.));
#6452=CARTESIAN_POINT('Origin',(6.5,0.,5.));
#6453=CARTESIAN_POINT('',(5.,3.,5.));
#6454=CARTESIAN_POINT('',(8.,3.,5.));
#6455=CARTESIAN_POINT('',(5.,3.,5.));
#6456=CARTESIAN_POINT('Origin',(6.5,-2.5,0.9));
#6457=CARTESIAN_POINT('',(6.17,-2.5,1.));
#6458=CARTESIAN_POINT('Origin',(6.5,-2.5,1.));
#6459=CARTESIAN_POINT('',(6.17,-2.5,0.9));
#6460=CARTESIAN_POINT('Origin',(6.5,2.5,0.9));
#6461=CARTESIAN_POINT('',(6.17,2.5,1.));
#6462=CARTESIAN_POINT('Origin',(6.5,2.5,1.));
#6463=CARTESIAN_POINT('',(6.17,2.5,0.9));
#6464=CARTESIAN_POINT('Origin',(6.5,0.,5.));
#6465=CARTESIAN_POINT('',(5.,-3.,5.));
#6466=CARTESIAN_POINT('',(5.,3.,5.));
#6467=CARTESIAN_POINT('',(5.,-3.,5.));
#6468=CARTESIAN_POINT('Origin',(6.5,0.,5.));
#6469=CARTESIAN_POINT('',(8.,3.,5.));
#6470=CARTESIAN_POINT('',(8.,-3.,5.));
#6471=CARTESIAN_POINT('',(8.,3.,5.));
#6472=CARTESIAN_POINT('Origin',(5.,3.,1.));
#6473=CARTESIAN_POINT('',(5.,3.,1.));
#6474=CARTESIAN_POINT('',(5.,3.,1.));
#6475=CARTESIAN_POINT('',(5.,-3.,1.));
#6476=CARTESIAN_POINT('',(5.,3.,1.));
#6477=CARTESIAN_POINT('',(5.,-3.,1.));
#6478=CARTESIAN_POINT('Origin',(8.,3.,1.));
#6479=CARTESIAN_POINT('',(8.,3.,1.));
#6480=CARTESIAN_POINT('',(8.,3.,1.));
#6481=CARTESIAN_POINT('',(8.,3.,1.));
#6482=CARTESIAN_POINT('Origin',(8.,-3.,1.));
#6483=CARTESIAN_POINT('',(8.,-3.,1.));
#6484=CARTESIAN_POINT('',(8.,-3.,1.));
#6485=CARTESIAN_POINT('',(8.,-3.,1.));
#6486=CARTESIAN_POINT('Origin',(5.,-3.,1.));
#6487=CARTESIAN_POINT('',(5.,-3.,1.));
#6488=CARTESIAN_POINT('Origin',(6.5,0.,1.));
#7300=UNCERTAINTY_MEASURE_WITH_UNIT(LENGTH_MEASURE(0.001),#7345,
'DISTANCE_ACCURACY_VALUE',
'Maximum model space distance between geometric entities at asserted c
onnectivities');
#7318=UNCERTAINTY_MEASURE_WITH_UNIT(LENGTH_MEASURE(0.001),#7345,
'DISTANCE_ACCURACY_VALUE',
'Maximum model space distance between geometric entities at asserted c
onnectivities');
#7326=(
GEOMETRIC_REPRESENTATION_CONTEXT(3)
GLOBAL_UNCERTAINTY_ASSIGNED_CONTEXT((#7300))
GLOBAL_UNIT_ASSIGNED_CONTEXT((#7345,#7347,#7348))
REPRESENTATION_CONTEXT('','3D')
);
#7344=(
GEOMETRIC_REPRESENTATION_CONTEXT(3)
GLOBAL_UNCERTAINTY_ASSIGNED_CONTEXT((#7318))
GLOBAL_UNIT_ASSIGNED_CONTEXT((#7345,#7347,#7348))
REPRESENTATION_CONTEXT('','3D')
);
#7345=(
LENGTH_UNIT()
NAMED_UNIT(*)
SI_UNIT(.CENTI.,.METRE.)
);
#7347=(
NAMED_UNIT(*)
PLANE_ANGLE_UNIT()
SI_UNIT($,.RADIAN.)
);
#7348=(
NAMED_UNIT(*)
SI_UNIT($,.STERADIAN.)
SOLID_ANGLE_UNIT()
);
#7356=SHAPE_DEFINITION_REPRESENTATION(#7381,#7447);
#7381=PRODUCT_DEFINITION_SHAPE('',$,#7473);
#7447=SHAPE_REPRESENTATION('',(#4499),#7326);
#7465=PRODUCT_DEFINITION_CONTEXT('part definition',#7542,'design');
#7473=PRODUCT_DEFINITION('V block','V block',#7498,#7465);
#7498=PRODUCT_DEFINITION_FORMATION('',$,#7551);
#7542=APPLICATION_CONTEXT(
'Core Data for Automotive Mechanical Design Process');
#7543=PRODUCT_CONTEXT('part definition',#7542,'mechanical');
#7551=PRODUCT('V block','V block','V block',(#7543));
#7604=COLOUR_RGB('Dark Blue',0.08,0.2,0.34);
#7605=FILL_AREA_STYLE_COLOUR('',#7604);
#7606=FILL_AREA_STYLE('',(#7605));
#7607=SURFACE_STYLE_FILL_AREA(#7606);
#7608=SURFACE_SIDE_STYLE('',(#7607));
#7609=SURFACE_STYLE_USAGE(.BOTH.,#7608);
#7610=PRESENTATION_STYLE_ASSIGNMENT((#7609));
ENDSEC;
END-ISO-10303-21;
